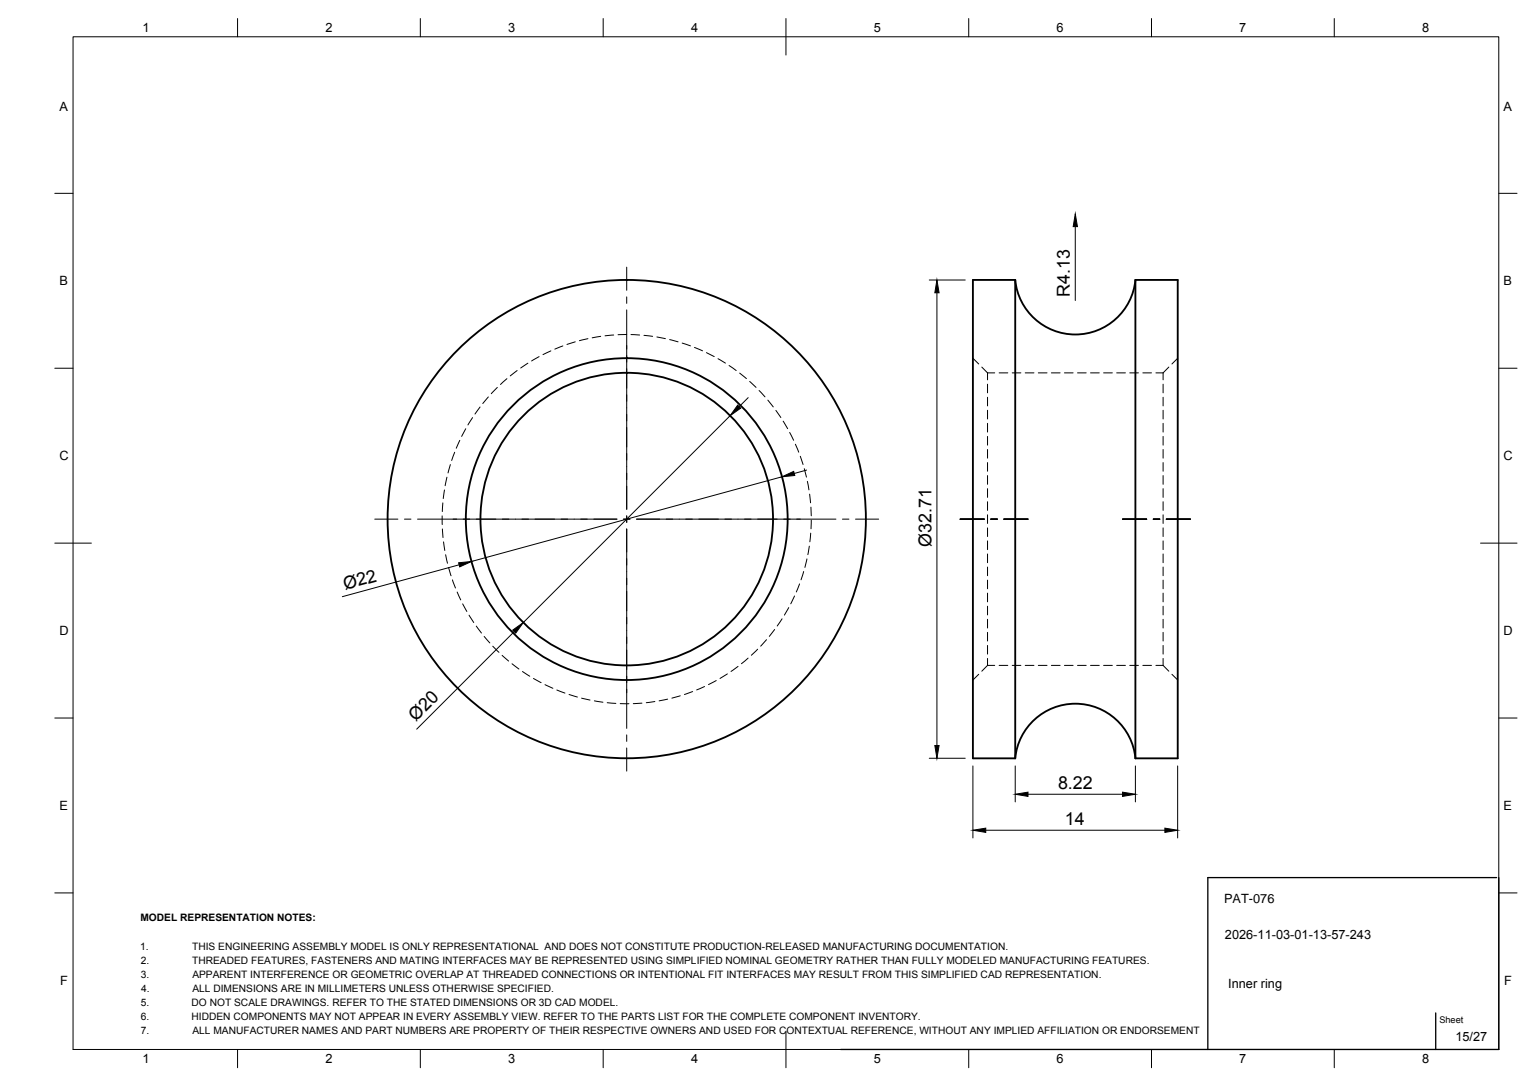
ISO-10303-21;
HEADER;
/* Generated by software containing ST-Developer
 * from STEP Tools, Inc. (www.steptools.com) 
 */

FILE_DESCRIPTION(
/* description */ ('Overhung pulley bearing cartridge'),
/* implementation_level */ '2;1');

FILE_NAME(
/* name */ 'Inner ring.step',
/* time_stamp */ '2026-10-28T03:22:33-07:00',
/* author */ (''),
/* organization */ (''),
/* preprocessor_version */ 'ST-DEVELOPER v20.2',
/* originating_system */ 'Autodesk Translation Framework v15.17.0.0',
/* authorisation */ '');

FILE_SCHEMA (('AUTOMOTIVE_DESIGN { 1 0 10303 214 3 1 1 }'));
ENDSEC;

DATA;
#10=MECHANICAL_DESIGN_GEOMETRIC_PRESENTATION_REPRESENTATION('',(#291),#10963);
#223=CONICAL_SURFACE('',#6124,1.05,0.785398163397449);
#224=CONICAL_SURFACE('',#6131,1.05,0.785398163397449);
#237=TOROIDAL_SURFACE('',#6113,1.675,0.412776);
#247=SHAPE_REPRESENTATION_RELATIONSHIP('SRR','None',#11068,#269);
#269=ADVANCED_BREP_SHAPE_REPRESENTATION('',(#321),#10948);
#291=STYLED_ITEM('',(#11253),#321);
#321=MANIFOLD_SOLID_BREP('Body1',#5658);
#396=FACE_BOUND('',#1060,.T.);
#397=FACE_BOUND('',#1063,.T.);
#491=PLANE('',#6126);
#492=PLANE('',#6129);
#671=FACE_OUTER_BOUND('',#1055,.T.);
#672=FACE_OUTER_BOUND('',#1056,.T.);
#673=FACE_OUTER_BOUND('',#1057,.T.);
#674=FACE_OUTER_BOUND('',#1058,.T.);
#675=FACE_OUTER_BOUND('',#1059,.T.);
#676=FACE_OUTER_BOUND('',#1061,.T.);
#677=FACE_OUTER_BOUND('',#1062,.T.);
#678=FACE_OUTER_BOUND('',#1064,.T.);
#1055=EDGE_LOOP('',(#4035,#4036,#4037,#4038,#4039,#4040));
#1056=EDGE_LOOP('',(#4041,#4042,#4043,#4044,#4045));
#1057=EDGE_LOOP('',(#4046,#4047,#4048,#4049));
#1058=EDGE_LOOP('',(#4050,#4051,#4052,#4053));
#1059=EDGE_LOOP('',(#4054));
#1060=EDGE_LOOP('',(#4055));
#1061=EDGE_LOOP('',(#4056,#4057,#4058,#4059,#4060));
#1062=EDGE_LOOP('',(#4061));
#1063=EDGE_LOOP('',(#4062));
#1064=EDGE_LOOP('',(#4063,#4064,#4065,#4066));
#1437=LINE('',#8991,#1779);
#1438=LINE('',#8997,#1780);
#1439=LINE('',#9001,#1781);
#1440=LINE('',#9007,#1782);
#1441=LINE('',#9012,#1783);
#1779=VECTOR('',#7187,1.63531);
#1780=VECTOR('',#7194,1.);
#1781=VECTOR('',#7199,1.05);
#1782=VECTOR('',#7208,1.63531);
#1783=VECTOR('',#7215,1.05);
#2094=CIRCLE('',#6114,1.63531);
#2095=CIRCLE('',#6115,1.63531);
#2096=CIRCLE('',#6116,0.412776);
#2097=CIRCLE('',#6117,1.63531);
#2098=CIRCLE('',#6118,1.63531);
#2099=CIRCLE('',#6120,1.63531);
#2100=CIRCLE('',#6122,1.);
#2101=CIRCLE('',#6123,1.);
#2102=CIRCLE('',#6125,1.1);
#2103=CIRCLE('',#6128,1.63531);
#2104=CIRCLE('',#6130,1.1);
#2509=VERTEX_POINT('',#8980);
#2510=VERTEX_POINT('',#8981);
#2511=VERTEX_POINT('',#8984);
#2512=VERTEX_POINT('',#8986);
#2513=VERTEX_POINT('',#8990);
#2514=VERTEX_POINT('',#8994);
#2515=VERTEX_POINT('',#8996);
#2516=VERTEX_POINT('',#9000);
#2517=VERTEX_POINT('',#9005);
#2518=VERTEX_POINT('',#9009);
#3087=EDGE_CURVE('',#2509,#2510,#2094,.T.);
#3088=EDGE_CURVE('',#2510,#2509,#2095,.T.);
#3089=EDGE_CURVE('',#2510,#2511,#2096,.T.);
#3090=EDGE_CURVE('',#2512,#2511,#2097,.T.);
#3091=EDGE_CURVE('',#2511,#2512,#2098,.T.);
#3092=EDGE_CURVE('',#2512,#2513,#1437,.T.);
#3093=EDGE_CURVE('',#2513,#2513,#2099,.T.);
#3094=EDGE_CURVE('',#2514,#2514,#2100,.T.);
#3095=EDGE_CURVE('',#2514,#2515,#1438,.T.);
#3096=EDGE_CURVE('',#2515,#2515,#2101,.T.);
#3097=EDGE_CURVE('',#2515,#2516,#1439,.T.);
#3098=EDGE_CURVE('',#2516,#2516,#2102,.T.);
#3099=EDGE_CURVE('',#2517,#2517,#2103,.T.);
#3100=EDGE_CURVE('',#2517,#2509,#1440,.T.);
#3101=EDGE_CURVE('',#2518,#2518,#2104,.T.);
#3102=EDGE_CURVE('',#2518,#2514,#1441,.T.);
#4035=ORIENTED_EDGE('',*,*,#3087,.F.);
#4036=ORIENTED_EDGE('',*,*,#3088,.F.);
#4037=ORIENTED_EDGE('',*,*,#3089,.T.);
#4038=ORIENTED_EDGE('',*,*,#3090,.F.);
#4039=ORIENTED_EDGE('',*,*,#3091,.F.);
#4040=ORIENTED_EDGE('',*,*,#3089,.F.);
#4041=ORIENTED_EDGE('',*,*,#3090,.T.);
#4042=ORIENTED_EDGE('',*,*,#3091,.T.);
#4043=ORIENTED_EDGE('',*,*,#3092,.T.);
#4044=ORIENTED_EDGE('',*,*,#3093,.T.);
#4045=ORIENTED_EDGE('',*,*,#3092,.F.);
#4046=ORIENTED_EDGE('',*,*,#3094,.T.);
#4047=ORIENTED_EDGE('',*,*,#3095,.T.);
#4048=ORIENTED_EDGE('',*,*,#3096,.F.);
#4049=ORIENTED_EDGE('',*,*,#3095,.F.);
#4050=ORIENTED_EDGE('',*,*,#3096,.T.);
#4051=ORIENTED_EDGE('',*,*,#3097,.T.);
#4052=ORIENTED_EDGE('',*,*,#3098,.F.);
#4053=ORIENTED_EDGE('',*,*,#3097,.F.);
#4054=ORIENTED_EDGE('',*,*,#3093,.F.);
#4055=ORIENTED_EDGE('',*,*,#3098,.T.);
#4056=ORIENTED_EDGE('',*,*,#3099,.F.);
#4057=ORIENTED_EDGE('',*,*,#3100,.T.);
#4058=ORIENTED_EDGE('',*,*,#3087,.T.);
#4059=ORIENTED_EDGE('',*,*,#3088,.T.);
#4060=ORIENTED_EDGE('',*,*,#3100,.F.);
#4061=ORIENTED_EDGE('',*,*,#3099,.T.);
#4062=ORIENTED_EDGE('',*,*,#3101,.F.);
#4063=ORIENTED_EDGE('',*,*,#3101,.T.);
#4064=ORIENTED_EDGE('',*,*,#3102,.T.);
#4065=ORIENTED_EDGE('',*,*,#3094,.F.);
#4066=ORIENTED_EDGE('',*,*,#3102,.F.);
#5204=CYLINDRICAL_SURFACE('',#6119,1.63531);
#5205=CYLINDRICAL_SURFACE('',#6121,1.);
#5206=CYLINDRICAL_SURFACE('',#6127,1.63531);
#5415=ADVANCED_FACE('',(#671),#237,.F.);
#5416=ADVANCED_FACE('',(#672),#5204,.T.);
#5417=ADVANCED_FACE('',(#673),#5205,.F.);
#5418=ADVANCED_FACE('',(#674),#223,.F.);
#5419=ADVANCED_FACE('',(#675,#396),#491,.T.);
#5420=ADVANCED_FACE('',(#676),#5206,.T.);
#5421=ADVANCED_FACE('',(#677,#397),#492,.T.);
#5422=ADVANCED_FACE('',(#678),#224,.F.);
#5658=CLOSED_SHELL('',(#5415,#5416,#5417,#5418,#5419,#5420,#5421,#5422));
#6112=AXIS2_PLACEMENT_3D('',#8978,#7171,#7172);
#6113=AXIS2_PLACEMENT_3D('',#8979,#7173,#7174);
#6114=AXIS2_PLACEMENT_3D('',#8982,#7175,#7176);
#6115=AXIS2_PLACEMENT_3D('',#8983,#7177,#7178);
#6116=AXIS2_PLACEMENT_3D('',#8985,#7179,#7180);
#6117=AXIS2_PLACEMENT_3D('',#8987,#7181,#7182);
#6118=AXIS2_PLACEMENT_3D('',#8988,#7183,#7184);
#6119=AXIS2_PLACEMENT_3D('',#8989,#7185,#7186);
#6120=AXIS2_PLACEMENT_3D('',#8992,#7188,#7189);
#6121=AXIS2_PLACEMENT_3D('',#8993,#7190,#7191);
#6122=AXIS2_PLACEMENT_3D('',#8995,#7192,#7193);
#6123=AXIS2_PLACEMENT_3D('',#8998,#7195,#7196);
#6124=AXIS2_PLACEMENT_3D('',#8999,#7197,#7198);
#6125=AXIS2_PLACEMENT_3D('',#9002,#7200,#7201);
#6126=AXIS2_PLACEMENT_3D('',#9003,#7202,#7203);
#6127=AXIS2_PLACEMENT_3D('',#9004,#7204,#7205);
#6128=AXIS2_PLACEMENT_3D('',#9006,#7206,#7207);
#6129=AXIS2_PLACEMENT_3D('',#9008,#7209,#7210);
#6130=AXIS2_PLACEMENT_3D('',#9010,#7211,#7212);
#6131=AXIS2_PLACEMENT_3D('',#9011,#7213,#7214);
#7171=DIRECTION('axis',(0.,0.,1.));
#7172=DIRECTION('refdir',(1.,0.,0.));
#7173=DIRECTION('center_axis',(0.,-1.,0.));
#7174=DIRECTION('ref_axis',(0.,0.,-1.));
#7175=DIRECTION('center_axis',(0.,-1.,0.));
#7176=DIRECTION('ref_axis',(1.,0.,0.));
#7177=DIRECTION('center_axis',(0.,-1.,0.));
#7178=DIRECTION('ref_axis',(1.,0.,0.));
#7179=DIRECTION('center_axis',(1.,0.,1.22464679914735E-16));
#7180=DIRECTION('ref_axis',(-1.22464679914735E-16,0.,1.));
#7181=DIRECTION('center_axis',(0.,1.,0.));
#7182=DIRECTION('ref_axis',(1.,0.,0.));
#7183=DIRECTION('center_axis',(0.,1.,0.));
#7184=DIRECTION('ref_axis',(1.,0.,0.));
#7185=DIRECTION('center_axis',(0.,-1.,0.));
#7186=DIRECTION('ref_axis',(1.,0.,0.));
#7187=DIRECTION('',(0.,1.,0.));
#7188=DIRECTION('center_axis',(0.,-1.,0.));
#7189=DIRECTION('ref_axis',(1.,0.,0.));
#7190=DIRECTION('center_axis',(0.,-1.,0.));
#7191=DIRECTION('ref_axis',(1.,0.,0.));
#7192=DIRECTION('center_axis',(0.,-1.,0.));
#7193=DIRECTION('ref_axis',(1.,0.,0.));
#7194=DIRECTION('',(0.,1.,0.));
#7195=DIRECTION('center_axis',(0.,-1.,0.));
#7196=DIRECTION('ref_axis',(1.,0.,0.));
#7197=DIRECTION('center_axis',(0.,1.,0.));
#7198=DIRECTION('ref_axis',(1.,0.,0.));
#7199=DIRECTION('',(-0.707106781186548,0.707106781186547,-8.65956056235494E-17));
#7200=DIRECTION('center_axis',(0.,-1.,0.));
#7201=DIRECTION('ref_axis',(1.,0.,0.));
#7202=DIRECTION('center_axis',(0.,1.,0.));
#7203=DIRECTION('ref_axis',(0.,0.,1.));
#7204=DIRECTION('center_axis',(0.,-1.,0.));
#7205=DIRECTION('ref_axis',(1.,0.,0.));
#7206=DIRECTION('center_axis',(0.,-1.,0.));
#7207=DIRECTION('ref_axis',(1.,0.,0.));
#7208=DIRECTION('',(0.,1.,0.));
#7209=DIRECTION('center_axis',(0.,-1.,0.));
#7210=DIRECTION('ref_axis',(0.,0.,-1.));
#7211=DIRECTION('center_axis',(0.,-1.,0.));
#7212=DIRECTION('ref_axis',(1.,0.,0.));
#7213=DIRECTION('center_axis',(0.,-1.,0.));
#7214=DIRECTION('ref_axis',(1.,0.,0.));
#7215=DIRECTION('',(0.707106781186548,0.707106781186547,8.65956056235494E-17));
#8978=CARTESIAN_POINT('',(0.,0.,0.));
#8979=CARTESIAN_POINT('Origin',(0.,0.,0.));
#8980=CARTESIAN_POINT('',(-1.63531,-0.410863395882378,-2.00267715711366E-16));
#8981=CARTESIAN_POINT('',(-2.00267715711366E-16,-0.410863395882378,1.63531));
#8982=CARTESIAN_POINT('Origin',(0.,-0.410863395882378,0.));
#8983=CARTESIAN_POINT('Origin',(0.,-0.410863395882378,0.));
#8984=CARTESIAN_POINT('',(-2.00267715711366E-16,0.410863395882378,1.63531));
#8985=CARTESIAN_POINT('Origin',(-2.05128338857182E-16,0.,1.675));
#8986=CARTESIAN_POINT('',(-1.63531,0.410863395882378,2.00267715711366E-16));
#8987=CARTESIAN_POINT('Origin',(0.,0.410863395882378,0.));
#8988=CARTESIAN_POINT('Origin',(0.,0.410863395882378,0.));
#8989=CARTESIAN_POINT('Origin',(0.,0.,0.));
#8990=CARTESIAN_POINT('',(-1.63531,0.7,-2.00267715711366E-16));
#8991=CARTESIAN_POINT('',(-1.63531,0.,-2.00267715711366E-16));
#8992=CARTESIAN_POINT('Origin',(0.,0.7,0.));
#8993=CARTESIAN_POINT('Origin',(0.,0.,0.));
#8994=CARTESIAN_POINT('',(-1.,-0.6,-1.22464679914735E-16));
#8995=CARTESIAN_POINT('Origin',(0.,-0.6,0.));
#8996=CARTESIAN_POINT('',(-1.,0.6,-1.22464679914735E-16));
#8997=CARTESIAN_POINT('',(-1.,0.,-1.22464679914735E-16));
#8998=CARTESIAN_POINT('Origin',(0.,0.6,0.));
#8999=CARTESIAN_POINT('Origin',(0.,0.65,0.));
#9000=CARTESIAN_POINT('',(-1.1,0.7,-1.34711147906209E-16));
#9001=CARTESIAN_POINT('',(-1.05,0.65,-1.28587913910472E-16));
#9002=CARTESIAN_POINT('Origin',(0.,0.7,0.));
#9003=CARTESIAN_POINT('Origin',(1.63531,0.7,0.));
#9004=CARTESIAN_POINT('Origin',(0.,0.,0.));
#9005=CARTESIAN_POINT('',(-1.63531,-0.7,-2.00267715711366E-16));
#9006=CARTESIAN_POINT('Origin',(0.,-0.7,0.));
#9007=CARTESIAN_POINT('',(-1.63531,0.,-2.00267715711366E-16));
#9008=CARTESIAN_POINT('Origin',(1.1,-0.7,0.));
#9009=CARTESIAN_POINT('',(-1.1,-0.7,-1.34711147906209E-16));
#9010=CARTESIAN_POINT('Origin',(0.,-0.7,0.));
#9011=CARTESIAN_POINT('Origin',(0.,-0.65,0.));
#9012=CARTESIAN_POINT('',(-1.05,-0.65,-1.28587913910472E-16));
#10921=UNCERTAINTY_MEASURE_WITH_UNIT(LENGTH_MEASURE(0.001),#10964,
'DISTANCE_ACCURACY_VALUE',
'Maximum model space distance between geometric entities at asserted c
onnectivities');
#10936=UNCERTAINTY_MEASURE_WITH_UNIT(LENGTH_MEASURE(0.001),#10964,
'DISTANCE_ACCURACY_VALUE',
'Maximum model space distance between geometric entities at asserted c
onnectivities');
#10948=(
GEOMETRIC_REPRESENTATION_CONTEXT(3)
GLOBAL_UNCERTAINTY_ASSIGNED_CONTEXT((#10921))
GLOBAL_UNIT_ASSIGNED_CONTEXT((#10964,#10966,#10967))
REPRESENTATION_CONTEXT('','3D')
);
#10963=(
GEOMETRIC_REPRESENTATION_CONTEXT(3)
GLOBAL_UNCERTAINTY_ASSIGNED_CONTEXT((#10936))
GLOBAL_UNIT_ASSIGNED_CONTEXT((#10964,#10966,#10967))
REPRESENTATION_CONTEXT('','3D')
);
#10964=(
LENGTH_UNIT()
NAMED_UNIT(*)
SI_UNIT(.CENTI.,.METRE.)
);
#10966=(
NAMED_UNIT(*)
PLANE_ANGLE_UNIT()
SI_UNIT($,.RADIAN.)
);
#10967=(
NAMED_UNIT(*)
SI_UNIT($,.STERADIAN.)
SOLID_ANGLE_UNIT()
);
#10979=SHAPE_DEFINITION_REPRESENTATION(#11005,#11068);
#11005=PRODUCT_DEFINITION_SHAPE('',$,#11095);
#11068=SHAPE_REPRESENTATION('',(#6112),#10948);
#11083=PRODUCT_DEFINITION_CONTEXT('part definition',#11163,'design');
#11095=PRODUCT_DEFINITION('Inner ring','Inner ring',#11121,#11083);
#11121=PRODUCT_DEFINITION_FORMATION('',$,#11176);
#11163=APPLICATION_CONTEXT(
'Core Data for Automotive Mechanical Design Process');
#11164=PRODUCT_CONTEXT('part definition',#11163,'mechanical');
#11176=PRODUCT('Inner ring','Inner ring','Inner ring',(#11164));
#11247=COLOUR_RGB('Grey',0.48,0.52,0.57);
#11248=FILL_AREA_STYLE_COLOUR('',#11247);
#11249=FILL_AREA_STYLE('',(#11248));
#11250=SURFACE_STYLE_FILL_AREA(#11249);
#11251=SURFACE_SIDE_STYLE('',(#11250));
#11252=SURFACE_STYLE_USAGE(.BOTH.,#11251);
#11253=PRESENTATION_STYLE_ASSIGNMENT((#11252));
ENDSEC;
END-ISO-10303-21;
